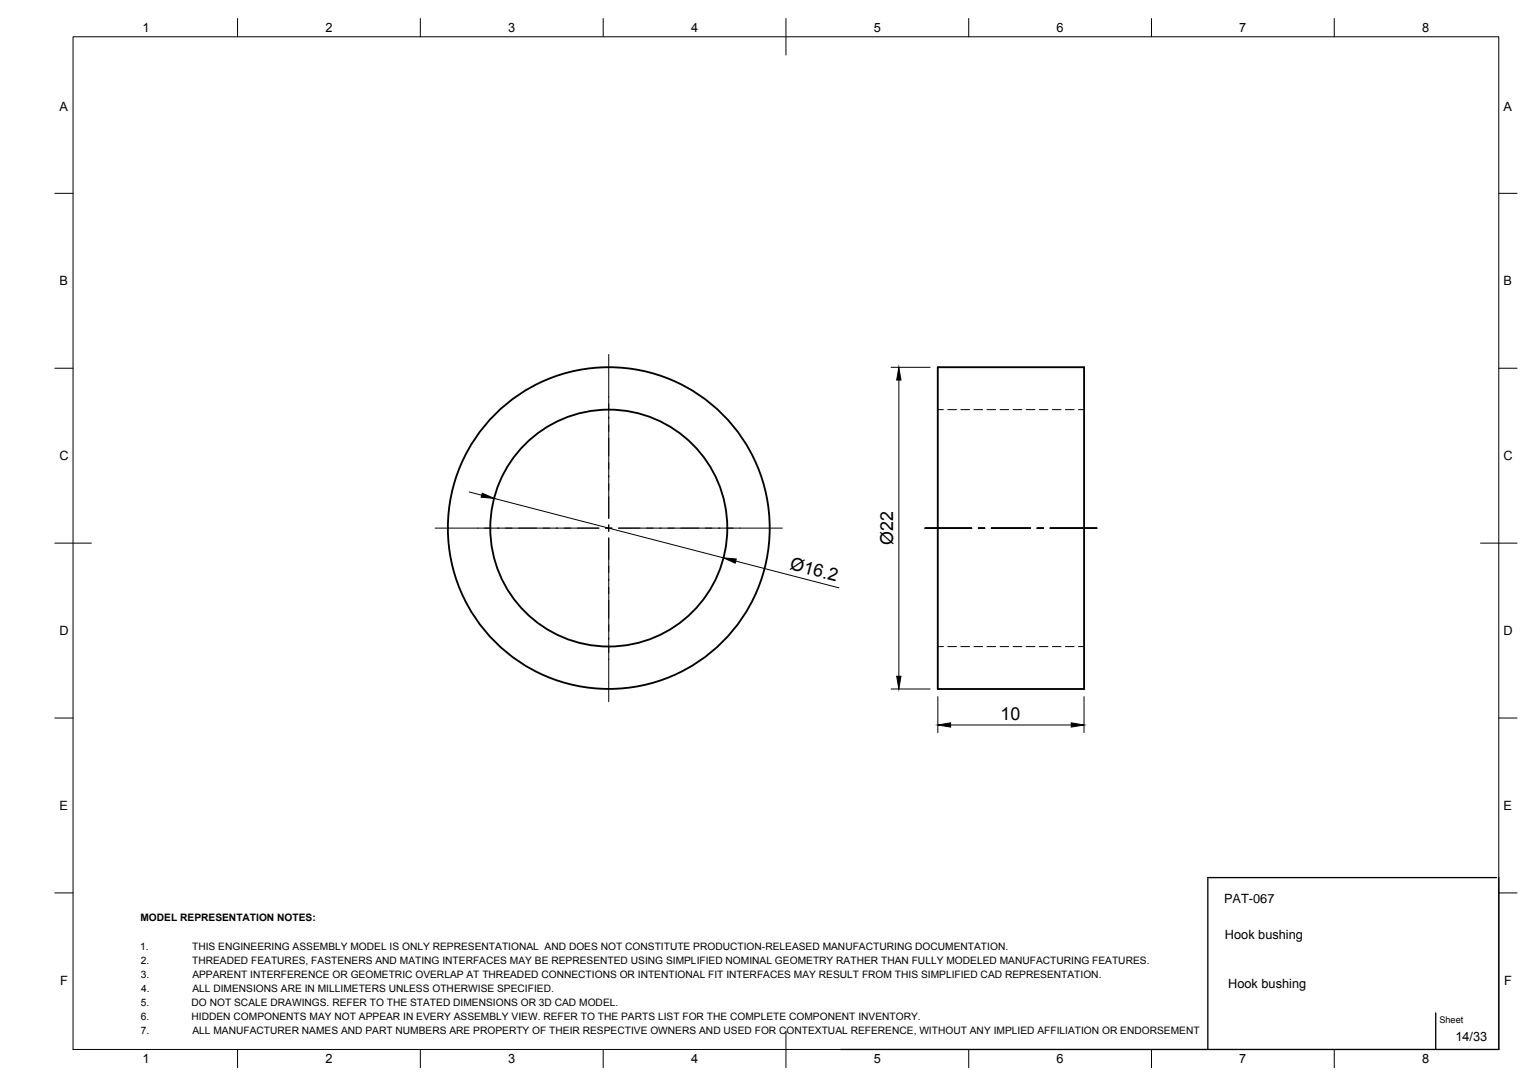
ISO-10303-21;
HEADER;
/* Generated by software containing ST-Developer
 * from STEP Tools, Inc. (www.steptools.com) 
 */

FILE_DESCRIPTION(
/* description */ ('Lifting hook block with sheave'),
/* implementation_level */ '2;1');

FILE_NAME(
/* name */ 'Hook bushing.step',
/* time_stamp */ '2026-10-28T03:23:54-07:00',
/* author */ (''),
/* organization */ (''),
/* preprocessor_version */ 'ST-DEVELOPER v20.2',
/* originating_system */ 'Autodesk Translation Framework v15.17.0.0',
/* authorisation */ '');

FILE_SCHEMA (('AUTOMOTIVE_DESIGN { 1 0 10303 214 3 1 1 }'));
ENDSEC;

DATA;
#10=MECHANICAL_DESIGN_GEOMETRIC_PRESENTATION_REPRESENTATION('',(#360),#9391);
#300=SHAPE_REPRESENTATION_RELATIONSHIP('SRR','None',#9531,#330);
#330=ADVANCED_BREP_SHAPE_REPRESENTATION('',(#398),#9366);
#360=STYLED_ITEM('',(#9745),#398);
#398=MANIFOLD_SOLID_BREP('Body1',#4896);
#534=LINE('',#8009,#822);
#535=LINE('',#8015,#823);
#822=VECTOR('',#6439,0.81);
#823=VECTOR('',#6446,1.1);
#1042=CYLINDRICAL_SURFACE('',#5457,0.81);
#1043=CYLINDRICAL_SURFACE('',#5460,1.1);
#1153=FACE_BOUND('',#1646,.T.);
#1154=FACE_BOUND('',#1648,.T.);
#1308=FACE_OUTER_BOUND('',#1643,.T.);
#1309=FACE_OUTER_BOUND('',#1644,.T.);
#1310=FACE_OUTER_BOUND('',#1645,.T.);
#1311=FACE_OUTER_BOUND('',#1647,.T.);
#1643=EDGE_LOOP('',(#3650,#3651,#3652,#3653));
#1644=EDGE_LOOP('',(#3654,#3655,#3656,#3657));
#1645=EDGE_LOOP('',(#3658));
#1646=EDGE_LOOP('',(#3659));
#1647=EDGE_LOOP('',(#3660));
#1648=EDGE_LOOP('',(#3661));
#2015=CIRCLE('',#5458,0.81);
#2016=CIRCLE('',#5459,0.81);
#2017=CIRCLE('',#5461,1.1);
#2018=CIRCLE('',#5462,1.1);
#2348=VERTEX_POINT('',#8006);
#2349=VERTEX_POINT('',#8008);
#2350=VERTEX_POINT('',#8012);
#2351=VERTEX_POINT('',#8014);
#2829=EDGE_CURVE('',#2348,#2348,#2015,.T.);
#2830=EDGE_CURVE('',#2348,#2349,#534,.T.);
#2831=EDGE_CURVE('',#2349,#2349,#2016,.T.);
#2832=EDGE_CURVE('',#2350,#2350,#2017,.T.);
#2833=EDGE_CURVE('',#2350,#2351,#535,.T.);
#2834=EDGE_CURVE('',#2351,#2351,#2018,.T.);
#3650=ORIENTED_EDGE('',*,*,#2829,.F.);
#3651=ORIENTED_EDGE('',*,*,#2830,.T.);
#3652=ORIENTED_EDGE('',*,*,#2831,.T.);
#3653=ORIENTED_EDGE('',*,*,#2830,.F.);
#3654=ORIENTED_EDGE('',*,*,#2832,.F.);
#3655=ORIENTED_EDGE('',*,*,#2833,.T.);
#3656=ORIENTED_EDGE('',*,*,#2834,.T.);
#3657=ORIENTED_EDGE('',*,*,#2833,.F.);
#3658=ORIENTED_EDGE('',*,*,#2832,.T.);
#3659=ORIENTED_EDGE('',*,*,#2829,.T.);
#3660=ORIENTED_EDGE('',*,*,#2834,.F.);
#3661=ORIENTED_EDGE('',*,*,#2831,.F.);
#4496=PLANE('',#5463);
#4497=PLANE('',#5464);
#4684=ADVANCED_FACE('',(#1308),#1042,.F.);
#4685=ADVANCED_FACE('',(#1309),#1043,.T.);
#4686=ADVANCED_FACE('',(#1310,#1153),#4496,.T.);
#4687=ADVANCED_FACE('',(#1311,#1154),#4497,.F.);
#4896=CLOSED_SHELL('',(#4684,#4685,#4686,#4687));
#5456=AXIS2_PLACEMENT_3D('',#8004,#6433,#6434);
#5457=AXIS2_PLACEMENT_3D('',#8005,#6435,#6436);
#5458=AXIS2_PLACEMENT_3D('',#8007,#6437,#6438);
#5459=AXIS2_PLACEMENT_3D('',#8010,#6440,#6441);
#5460=AXIS2_PLACEMENT_3D('',#8011,#6442,#6443);
#5461=AXIS2_PLACEMENT_3D('',#8013,#6444,#6445);
#5462=AXIS2_PLACEMENT_3D('',#8016,#6447,#6448);
#5463=AXIS2_PLACEMENT_3D('',#8017,#6449,#6450);
#5464=AXIS2_PLACEMENT_3D('',#8018,#6451,#6452);
#6433=DIRECTION('axis',(0.,0.,1.));
#6434=DIRECTION('refdir',(1.,0.,0.));
#6435=DIRECTION('center_axis',(0.,0.,1.));
#6436=DIRECTION('ref_axis',(1.,0.,0.));
#6437=DIRECTION('center_axis',(0.,0.,-1.));
#6438=DIRECTION('ref_axis',(1.,0.,0.));
#6439=DIRECTION('',(0.,0.,-1.));
#6440=DIRECTION('center_axis',(0.,0.,-1.));
#6441=DIRECTION('ref_axis',(1.,0.,0.));
#6442=DIRECTION('center_axis',(0.,0.,1.));
#6443=DIRECTION('ref_axis',(1.,0.,0.));
#6444=DIRECTION('center_axis',(0.,0.,1.));
#6445=DIRECTION('ref_axis',(1.,0.,0.));
#6446=DIRECTION('',(0.,0.,-1.));
#6447=DIRECTION('center_axis',(0.,0.,1.));
#6448=DIRECTION('ref_axis',(1.,0.,0.));
#6449=DIRECTION('center_axis',(0.,0.,1.));
#6450=DIRECTION('ref_axis',(1.,0.,0.));
#6451=DIRECTION('center_axis',(0.,0.,1.));
#6452=DIRECTION('ref_axis',(1.,0.,0.));
#8004=CARTESIAN_POINT('',(0.,0.,0.));
#8005=CARTESIAN_POINT('Origin',(0.,0.,4.5));
#8006=CARTESIAN_POINT('',(-0.81,-9.91963907309356E-17,5.5));
#8007=CARTESIAN_POINT('Origin',(0.,0.,5.5));
#8008=CARTESIAN_POINT('',(-0.81,-9.91963907309356E-17,4.5));
#8009=CARTESIAN_POINT('',(-0.81,-9.91963907309356E-17,4.5));
#8010=CARTESIAN_POINT('Origin',(0.,0.,4.5));
#8011=CARTESIAN_POINT('Origin',(0.,0.,4.5));
#8012=CARTESIAN_POINT('',(-1.1,-1.34711147906209E-16,5.5));
#8013=CARTESIAN_POINT('Origin',(0.,0.,5.5));
#8014=CARTESIAN_POINT('',(-1.1,-1.34711147906209E-16,4.5));
#8015=CARTESIAN_POINT('',(-1.1,-1.34711147906209E-16,4.5));
#8016=CARTESIAN_POINT('Origin',(0.,0.,4.5));
#8017=CARTESIAN_POINT('Origin',(0.,0.,5.5));
#8018=CARTESIAN_POINT('Origin',(0.,0.,4.5));
#9329=UNCERTAINTY_MEASURE_WITH_UNIT(LENGTH_MEASURE(0.001),#9392,
'DISTANCE_ACCURACY_VALUE',
'Maximum model space distance between geometric entities at asserted c
onnectivities');
#9354=UNCERTAINTY_MEASURE_WITH_UNIT(LENGTH_MEASURE(0.001),#9392,
'DISTANCE_ACCURACY_VALUE',
'Maximum model space distance between geometric entities at asserted c
onnectivities');
#9366=(
GEOMETRIC_REPRESENTATION_CONTEXT(3)
GLOBAL_UNCERTAINTY_ASSIGNED_CONTEXT((#9329))
GLOBAL_UNIT_ASSIGNED_CONTEXT((#9392,#9394,#9395))
REPRESENTATION_CONTEXT('','3D')
);
#9391=(
GEOMETRIC_REPRESENTATION_CONTEXT(3)
GLOBAL_UNCERTAINTY_ASSIGNED_CONTEXT((#9354))
GLOBAL_UNIT_ASSIGNED_CONTEXT((#9392,#9394,#9395))
REPRESENTATION_CONTEXT('','3D')
);
#9392=(
LENGTH_UNIT()
NAMED_UNIT(*)
SI_UNIT(.CENTI.,.METRE.)
);
#9394=(
NAMED_UNIT(*)
PLANE_ANGLE_UNIT()
SI_UNIT($,.RADIAN.)
);
#9395=(
NAMED_UNIT(*)
SI_UNIT($,.STERADIAN.)
SOLID_ANGLE_UNIT()
);
#9407=SHAPE_DEFINITION_REPRESENTATION(#9443,#9531);
#9443=PRODUCT_DEFINITION_SHAPE('',$,#9568);
#9531=SHAPE_REPRESENTATION('',(#5456),#9366);
#9556=PRODUCT_DEFINITION_CONTEXT('part definition',#9666,'design');
#9568=PRODUCT_DEFINITION('Hook bushing','Hook bushing',#9604,#9556);
#9604=PRODUCT_DEFINITION_FORMATION('',$,#9679);
#9666=APPLICATION_CONTEXT(
'Core Data for Automotive Mechanical Design Process');
#9667=PRODUCT_CONTEXT('part definition',#9666,'mechanical');
#9679=PRODUCT('Hook bushing','Hook bushing','Hook bushing',(#9667));
#9739=COLOUR_RGB('Light Blue',0.38,0.62,0.78);
#9740=FILL_AREA_STYLE_COLOUR('',#9739);
#9741=FILL_AREA_STYLE('',(#9740));
#9742=SURFACE_STYLE_FILL_AREA(#9741);
#9743=SURFACE_SIDE_STYLE('',(#9742));
#9744=SURFACE_STYLE_USAGE(.BOTH.,#9743);
#9745=PRESENTATION_STYLE_ASSIGNMENT((#9744));
ENDSEC;
END-ISO-10303-21;
